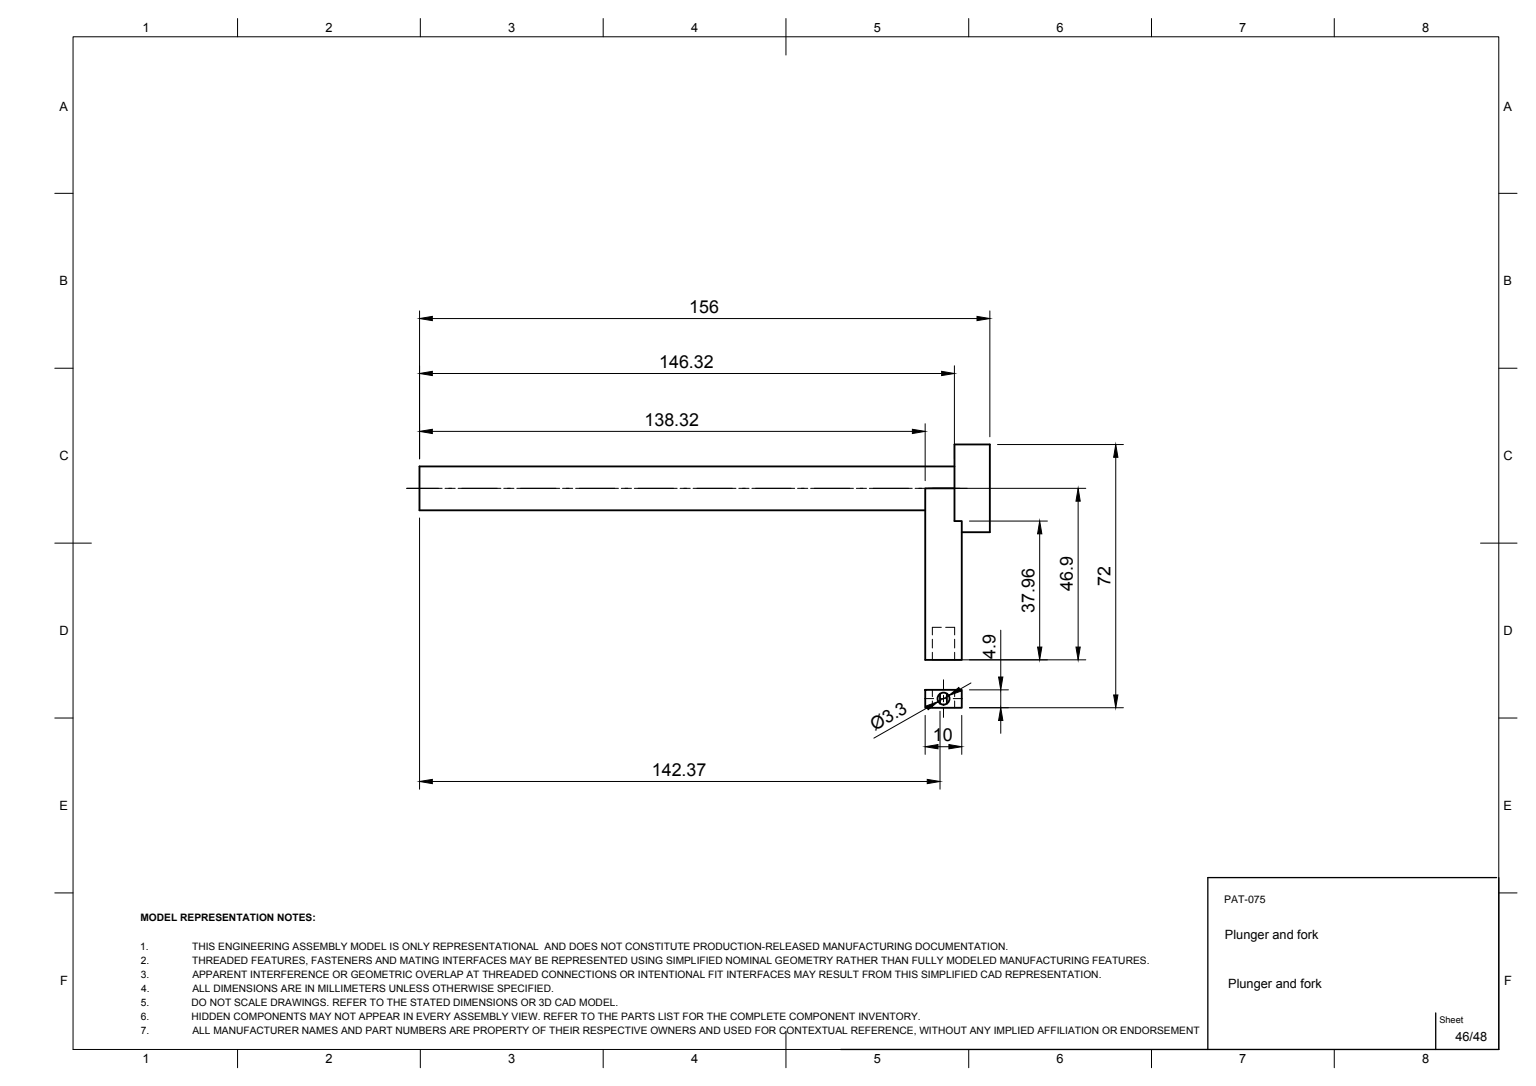
ISO-10303-21;
HEADER;
/* Generated by software containing ST-Developer
 * from STEP Tools, Inc. (www.steptools.com) 
 */

FILE_DESCRIPTION(
/* description */ ('Over-Centre Plunger Toggle Clamp on Slotted Fixture Frame'),
/* implementation_level */ '2;1');

FILE_NAME(
/* name */ 
'Plunger and fork.step',
/* time_stamp */ '2026-10-28T03:23:24-07:00',
/* author */ (''),
/* organization */ (''),
/* preprocessor_version */ 'ST-DEVELOPER v20.2',
/* originating_system */ 'Autodesk Translation Framework v15.17.0.0',
/* authorisation */ '');

FILE_SCHEMA (('AUTOMOTIVE_DESIGN { 1 0 10303 214 3 1 1 }'));
ENDSEC;

DATA;
#10=MECHANICAL_DESIGN_GEOMETRIC_PRESENTATION_REPRESENTATION('',(#559,#560),#15212);
#377=B_SPLINE_CURVE_WITH_KNOTS('',3,(#14965,#14966,#14967,#14968,#14969,
#14970,#14971,#14972,#14973,#14974),.UNSPECIFIED.,.F.,.F.,(4,2,2,2,4),(0.66642709076087,
0.700624974512804,0.764181514210609,0.827738053908413,0.861935937660348),
 .UNSPECIFIED.);
#378=B_SPLINE_CURVE_WITH_KNOTS('',3,(#14982,#14983,#14984,#14985,#14986,
#14987,#14988,#14989,#14990,#14991),.UNSPECIFIED.,.F.,.F.,(4,2,2,2,4),(0.156972747953797,
0.191170631705732,0.254727171403536,0.318283711101341,0.352481594853276),
 .UNSPECIFIED.);
#467=SHAPE_REPRESENTATION_RELATIONSHIP('SRR','None',#15446,#509);
#509=ADVANCED_BREP_SHAPE_REPRESENTATION('',(#606,#607),#15208);
#559=STYLED_ITEM('',(#15733),#606);
#560=STYLED_ITEM('',(#15733),#607);
#606=MANIFOLD_SOLID_BREP('Body1',#8295);
#607=MANIFOLD_SOLID_BREP('Body2',#8296);
#776=FACE_BOUND('',#2183,.T.);
#777=FACE_BOUND('',#2199,.T.);
#778=FACE_BOUND('',#2201,.T.);
#779=FACE_BOUND('',#2206,.T.);
#780=FACE_BOUND('',#2208,.T.);
#1054=PLANE('',#9677);
#1055=PLANE('',#9678);
#1056=PLANE('',#9679);
#1057=PLANE('',#9680);
#1058=PLANE('',#9682);
#1059=PLANE('',#9683);
#1060=PLANE('',#9684);
#1061=PLANE('',#9685);
#1062=PLANE('',#9690);
#1063=PLANE('',#9695);
#1064=PLANE('',#9696);
#1065=PLANE('',#9697);
#1066=PLANE('',#9703);
#1067=PLANE('',#9707);
#1068=PLANE('',#9708);
#1069=PLANE('',#9709);
#1070=PLANE('',#9710);
#1071=PLANE('',#9711);
#1072=PLANE('',#9712);
#1529=FACE_OUTER_BOUND('',#2180,.T.);
#1530=FACE_OUTER_BOUND('',#2181,.T.);
#1531=FACE_OUTER_BOUND('',#2182,.T.);
#1532=FACE_OUTER_BOUND('',#2184,.T.);
#1533=FACE_OUTER_BOUND('',#2185,.T.);
#1534=FACE_OUTER_BOUND('',#2186,.T.);
#1535=FACE_OUTER_BOUND('',#2187,.T.);
#1536=FACE_OUTER_BOUND('',#2188,.T.);
#1537=FACE_OUTER_BOUND('',#2189,.T.);
#1538=FACE_OUTER_BOUND('',#2190,.T.);
#1539=FACE_OUTER_BOUND('',#2191,.T.);
#1540=FACE_OUTER_BOUND('',#2192,.T.);
#1541=FACE_OUTER_BOUND('',#2193,.T.);
#1542=FACE_OUTER_BOUND('',#2194,.T.);
#1543=FACE_OUTER_BOUND('',#2195,.T.);
#1544=FACE_OUTER_BOUND('',#2196,.T.);
#1545=FACE_OUTER_BOUND('',#2197,.T.);
#1546=FACE_OUTER_BOUND('',#2198,.T.);
#1547=FACE_OUTER_BOUND('',#2200,.T.);
#1548=FACE_OUTER_BOUND('',#2202,.T.);
#1549=FACE_OUTER_BOUND('',#2203,.T.);
#1550=FACE_OUTER_BOUND('',#2204,.T.);
#1551=FACE_OUTER_BOUND('',#2205,.T.);
#1552=FACE_OUTER_BOUND('',#2207,.T.);
#2180=EDGE_LOOP('',(#7437,#7438,#7439,#7440));
#2181=EDGE_LOOP('',(#7441));
#2182=EDGE_LOOP('',(#7442,#7443,#7444,#7445));
#2183=EDGE_LOOP('',(#7446));
#2184=EDGE_LOOP('',(#7447,#7448,#7449,#7450,#7451,#7452));
#2185=EDGE_LOOP('',(#7453,#7454,#7455,#7456));
#2186=EDGE_LOOP('',(#7457,#7458,#7459,#7460,#7461,#7462));
#2187=EDGE_LOOP('',(#7463,#7464,#7465,#7466));
#2188=EDGE_LOOP('',(#7467,#7468,#7469,#7470));
#2189=EDGE_LOOP('',(#7471,#7472,#7473,#7474,#7475,#7476));
#2190=EDGE_LOOP('',(#7477,#7478,#7479,#7480,#7481,#7482,#7483));
#2191=EDGE_LOOP('',(#7484,#7485,#7486,#7487,#7488,#7489,#7490));
#2192=EDGE_LOOP('',(#7491,#7492,#7493,#7494,#7495,#7496,#7497,#7498));
#2193=EDGE_LOOP('',(#7499));
#2194=EDGE_LOOP('',(#7500));
#2195=EDGE_LOOP('',(#7501,#7502));
#2196=EDGE_LOOP('',(#7503,#7504,#7505,#7506,#7507,#7508,#7509,#7510));
#2197=EDGE_LOOP('',(#7511,#7512,#7513));
#2198=EDGE_LOOP('',(#7514,#7515,#7516,#7517));
#2199=EDGE_LOOP('',(#7518,#7519,#7520,#7521));
#2200=EDGE_LOOP('',(#7522,#7523,#7524,#7525));
#2201=EDGE_LOOP('',(#7526));
#2202=EDGE_LOOP('',(#7527,#7528,#7529,#7530));
#2203=EDGE_LOOP('',(#7531,#7532,#7533,#7534));
#2204=EDGE_LOOP('',(#7535,#7536,#7537,#7538));
#2205=EDGE_LOOP('',(#7539,#7540,#7541,#7542));
#2206=EDGE_LOOP('',(#7543));
#2207=EDGE_LOOP('',(#7544,#7545,#7546,#7547));
#2208=EDGE_LOOP('',(#7548));
#2798=LINE('',#14895,#3428);
#2799=LINE('',#14901,#3429);
#2800=LINE('',#14903,#3430);
#2801=LINE('',#14905,#3431);
#2802=LINE('',#14906,#3432);
#2803=LINE('',#14909,#3433);
#2804=LINE('',#14911,#3434);
#2805=LINE('',#14913,#3435);
#2806=LINE('',#14915,#3436);
#2807=LINE('',#14916,#3437);
#2808=LINE('',#14919,#3438);
#2809=LINE('',#14923,#3439);
#2810=LINE('',#14925,#3440);
#2811=LINE('',#14927,#3441);
#2812=LINE('',#14928,#3442);
#2813=LINE('',#14932,#3443);
#2814=LINE('',#14933,#3444);
#2815=LINE('',#14934,#3445);
#2816=LINE('',#14937,#3446);
#2817=LINE('',#14939,#3447);
#2818=LINE('',#14940,#3448);
#2819=LINE('',#14946,#3449);
#2820=LINE('',#14954,#3450);
#2821=LINE('',#14961,#3451);
#2822=LINE('',#14978,#3452);
#2823=LINE('',#14993,#3453);
#2824=LINE('',#14998,#3454);
#2825=LINE('',#15003,#3455);
#2826=LINE('',#15005,#3456);
#2827=LINE('',#15007,#3457);
#2828=LINE('',#15008,#3458);
#2829=LINE('',#15012,#3459);
#2830=LINE('',#15013,#3460);
#2831=LINE('',#15014,#3461);
#2832=LINE('',#15017,#3462);
#2833=LINE('',#15018,#3463);
#2834=LINE('',#15021,#3464);
#2835=LINE('',#15022,#3465);
#2836=LINE('',#15024,#3466);
#3428=VECTOR('',#12147,0.305);
#3429=VECTOR('',#12154,1.);
#3430=VECTOR('',#12155,1.);
#3431=VECTOR('',#12156,1.);
#3432=VECTOR('',#12157,1.);
#3433=VECTOR('',#12160,1.);
#3434=VECTOR('',#12161,1.);
#3435=VECTOR('',#12162,1.);
#3436=VECTOR('',#12163,1.);
#3437=VECTOR('',#12164,1.);
#3438=VECTOR('',#12167,1.);
#3439=VECTOR('',#12172,1.);
#3440=VECTOR('',#12173,1.);
#3441=VECTOR('',#12174,1.);
#3442=VECTOR('',#12175,1.);
#3443=VECTOR('',#12178,1.);
#3444=VECTOR('',#12179,1.);
#3445=VECTOR('',#12180,1.);
#3446=VECTOR('',#12183,1.);
#3447=VECTOR('',#12184,1.);
#3448=VECTOR('',#12185,1.);
#3449=VECTOR('',#12194,0.6);
#3450=VECTOR('',#12205,1.2);
#3451=VECTOR('',#12214,1.);
#3452=VECTOR('',#12221,0.165);
#3453=VECTOR('',#12228,1.);
#3454=VECTOR('',#12233,0.305);
#3455=VECTOR('',#12238,1.);
#3456=VECTOR('',#12239,1.);
#3457=VECTOR('',#12240,1.);
#3458=VECTOR('',#12241,1.);
#3459=VECTOR('',#12244,1.);
#3460=VECTOR('',#12245,1.);
#3461=VECTOR('',#12246,1.);
#3462=VECTOR('',#12249,1.);
#3463=VECTOR('',#12250,1.);
#3464=VECTOR('',#12253,1.);
#3465=VECTOR('',#12254,1.);
#3466=VECTOR('',#12257,1.);
#3834=CIRCLE('',#9675,0.305);
#3835=CIRCLE('',#9676,0.305);
#3836=CIRCLE('',#9681,1.2);
#3837=CIRCLE('',#9686,0.6);
#3838=CIRCLE('',#9688,0.6);
#3839=CIRCLE('',#9689,0.6);
#3840=CIRCLE('',#9691,1.2);
#3841=CIRCLE('',#9692,1.2);
#3842=CIRCLE('',#9694,1.2);
#3843=CIRCLE('',#9698,0.165);
#3844=CIRCLE('',#9700,0.165);
#3845=CIRCLE('',#9701,0.165);
#3846=CIRCLE('',#9702,0.165);
#3847=CIRCLE('',#9705,0.305);
#3848=CIRCLE('',#9706,0.305);
#4486=VERTEX_POINT('',#14892);
#4487=VERTEX_POINT('',#14894);
#4488=VERTEX_POINT('',#14899);
#4489=VERTEX_POINT('',#14900);
#4490=VERTEX_POINT('',#14902);
#4491=VERTEX_POINT('',#14904);
#4492=VERTEX_POINT('',#14908);
#4493=VERTEX_POINT('',#14910);
#4494=VERTEX_POINT('',#14912);
#4495=VERTEX_POINT('',#14914);
#4496=VERTEX_POINT('',#14918);
#4497=VERTEX_POINT('',#14922);
#4498=VERTEX_POINT('',#14924);
#4499=VERTEX_POINT('',#14926);
#4500=VERTEX_POINT('',#14930);
#4501=VERTEX_POINT('',#14931);
#4502=VERTEX_POINT('',#14936);
#4503=VERTEX_POINT('',#14938);
#4504=VERTEX_POINT('',#14944);
#4505=VERTEX_POINT('',#14949);
#4506=VERTEX_POINT('',#14953);
#4507=VERTEX_POINT('',#14959);
#4508=VERTEX_POINT('',#14960);
#4509=VERTEX_POINT('',#14964);
#4510=VERTEX_POINT('',#14975);
#4511=VERTEX_POINT('',#14977);
#4512=VERTEX_POINT('',#14980);
#4513=VERTEX_POINT('',#14995);
#4514=VERTEX_POINT('',#14997);
#4515=VERTEX_POINT('',#15001);
#4516=VERTEX_POINT('',#15002);
#4517=VERTEX_POINT('',#15004);
#4518=VERTEX_POINT('',#15006);
#4519=VERTEX_POINT('',#15010);
#4520=VERTEX_POINT('',#15011);
#4521=VERTEX_POINT('',#15016);
#4522=VERTEX_POINT('',#15020);
#5479=EDGE_CURVE('',#4486,#4486,#3834,.T.);
#5480=EDGE_CURVE('',#4486,#4487,#2798,.T.);
#5481=EDGE_CURVE('',#4487,#4487,#3835,.T.);
#5482=EDGE_CURVE('',#4488,#4489,#2799,.T.);
#5483=EDGE_CURVE('',#4490,#4488,#2800,.T.);
#5484=EDGE_CURVE('',#4491,#4490,#2801,.T.);
#5485=EDGE_CURVE('',#4489,#4491,#2802,.T.);
#5486=EDGE_CURVE('',#4490,#4492,#2803,.T.);
#5487=EDGE_CURVE('',#4493,#4492,#2804,.T.);
#5488=EDGE_CURVE('',#4494,#4493,#2805,.T.);
#5489=EDGE_CURVE('',#4494,#4495,#2806,.T.);
#5490=EDGE_CURVE('',#4491,#4495,#2807,.T.);
#5491=EDGE_CURVE('',#4496,#4488,#2808,.T.);
#5492=EDGE_CURVE('',#4492,#4496,#3836,.T.);
#5493=EDGE_CURVE('',#4497,#4489,#2809,.T.);
#5494=EDGE_CURVE('',#4498,#4497,#2810,.T.);
#5495=EDGE_CURVE('',#4499,#4498,#2811,.T.);
#5496=EDGE_CURVE('',#4496,#4499,#2812,.T.);
#5497=EDGE_CURVE('',#4500,#4501,#2813,.T.);
#5498=EDGE_CURVE('',#4495,#4500,#2814,.T.);
#5499=EDGE_CURVE('',#4501,#4494,#2815,.T.);
#5500=EDGE_CURVE('',#4498,#4502,#2816,.T.);
#5501=EDGE_CURVE('',#4503,#4497,#2817,.T.);
#5502=EDGE_CURVE('',#4502,#4503,#2818,.T.);
#5503=EDGE_CURVE('',#4503,#4500,#3837,.T.);
#5504=EDGE_CURVE('',#4504,#4504,#3838,.T.);
#5505=EDGE_CURVE('',#4504,#4503,#2819,.T.);
#5506=EDGE_CURVE('',#4501,#4502,#3839,.T.);
#5507=EDGE_CURVE('',#4493,#4505,#3840,.T.);
#5508=EDGE_CURVE('',#4505,#4499,#3841,.T.);
#5509=EDGE_CURVE('',#4505,#4506,#2820,.T.);
#5510=EDGE_CURVE('',#4506,#4506,#3842,.T.);
#5511=EDGE_CURVE('',#4507,#4508,#2821,.T.);
#5512=EDGE_CURVE('',#4507,#4508,#3843,.T.);
#5513=EDGE_CURVE('',#4509,#4507,#377,.T.);
#5514=EDGE_CURVE('',#4510,#4509,#3844,.T.);
#5515=EDGE_CURVE('',#4510,#4511,#2822,.T.);
#5516=EDGE_CURVE('',#4511,#4511,#3845,.T.);
#5517=EDGE_CURVE('',#4512,#4510,#3846,.T.);
#5518=EDGE_CURVE('',#4508,#4512,#378,.T.);
#5519=EDGE_CURVE('',#4512,#4509,#2823,.T.);
#5520=EDGE_CURVE('',#4513,#4513,#3847,.T.);
#5521=EDGE_CURVE('',#4513,#4514,#2824,.T.);
#5522=EDGE_CURVE('',#4514,#4514,#3848,.T.);
#5523=EDGE_CURVE('',#4515,#4516,#2825,.T.);
#5524=EDGE_CURVE('',#4516,#4517,#2826,.T.);
#5525=EDGE_CURVE('',#4518,#4517,#2827,.T.);
#5526=EDGE_CURVE('',#4515,#4518,#2828,.T.);
#5527=EDGE_CURVE('',#4519,#4520,#2829,.T.);
#5528=EDGE_CURVE('',#4520,#4515,#2830,.T.);
#5529=EDGE_CURVE('',#4519,#4518,#2831,.T.);
#5530=EDGE_CURVE('',#4521,#4519,#2832,.T.);
#5531=EDGE_CURVE('',#4517,#4521,#2833,.T.);
#5532=EDGE_CURVE('',#4520,#4522,#2834,.T.);
#5533=EDGE_CURVE('',#4516,#4522,#2835,.T.);
#5534=EDGE_CURVE('',#4522,#4521,#2836,.T.);
#7437=ORIENTED_EDGE('',*,*,#5479,.F.);
#7438=ORIENTED_EDGE('',*,*,#5480,.T.);
#7439=ORIENTED_EDGE('',*,*,#5481,.T.);
#7440=ORIENTED_EDGE('',*,*,#5480,.F.);
#7441=ORIENTED_EDGE('',*,*,#5481,.F.);
#7442=ORIENTED_EDGE('',*,*,#5482,.F.);
#7443=ORIENTED_EDGE('',*,*,#5483,.F.);
#7444=ORIENTED_EDGE('',*,*,#5484,.F.);
#7445=ORIENTED_EDGE('',*,*,#5485,.F.);
#7446=ORIENTED_EDGE('',*,*,#5479,.T.);
#7447=ORIENTED_EDGE('',*,*,#5484,.T.);
#7448=ORIENTED_EDGE('',*,*,#5486,.T.);
#7449=ORIENTED_EDGE('',*,*,#5487,.F.);
#7450=ORIENTED_EDGE('',*,*,#5488,.F.);
#7451=ORIENTED_EDGE('',*,*,#5489,.T.);
#7452=ORIENTED_EDGE('',*,*,#5490,.F.);
#7453=ORIENTED_EDGE('',*,*,#5483,.T.);
#7454=ORIENTED_EDGE('',*,*,#5491,.F.);
#7455=ORIENTED_EDGE('',*,*,#5492,.F.);
#7456=ORIENTED_EDGE('',*,*,#5486,.F.);
#7457=ORIENTED_EDGE('',*,*,#5482,.T.);
#7458=ORIENTED_EDGE('',*,*,#5493,.F.);
#7459=ORIENTED_EDGE('',*,*,#5494,.F.);
#7460=ORIENTED_EDGE('',*,*,#5495,.F.);
#7461=ORIENTED_EDGE('',*,*,#5496,.F.);
#7462=ORIENTED_EDGE('',*,*,#5491,.T.);
#7463=ORIENTED_EDGE('',*,*,#5497,.F.);
#7464=ORIENTED_EDGE('',*,*,#5498,.F.);
#7465=ORIENTED_EDGE('',*,*,#5489,.F.);
#7466=ORIENTED_EDGE('',*,*,#5499,.F.);
#7467=ORIENTED_EDGE('',*,*,#5500,.F.);
#7468=ORIENTED_EDGE('',*,*,#5494,.T.);
#7469=ORIENTED_EDGE('',*,*,#5501,.F.);
#7470=ORIENTED_EDGE('',*,*,#5502,.F.);
#7471=ORIENTED_EDGE('',*,*,#5485,.T.);
#7472=ORIENTED_EDGE('',*,*,#5490,.T.);
#7473=ORIENTED_EDGE('',*,*,#5498,.T.);
#7474=ORIENTED_EDGE('',*,*,#5503,.F.);
#7475=ORIENTED_EDGE('',*,*,#5501,.T.);
#7476=ORIENTED_EDGE('',*,*,#5493,.T.);
#7477=ORIENTED_EDGE('',*,*,#5504,.F.);
#7478=ORIENTED_EDGE('',*,*,#5505,.T.);
#7479=ORIENTED_EDGE('',*,*,#5503,.T.);
#7480=ORIENTED_EDGE('',*,*,#5497,.T.);
#7481=ORIENTED_EDGE('',*,*,#5506,.T.);
#7482=ORIENTED_EDGE('',*,*,#5502,.T.);
#7483=ORIENTED_EDGE('',*,*,#5505,.F.);
#7484=ORIENTED_EDGE('',*,*,#5495,.T.);
#7485=ORIENTED_EDGE('',*,*,#5500,.T.);
#7486=ORIENTED_EDGE('',*,*,#5506,.F.);
#7487=ORIENTED_EDGE('',*,*,#5499,.T.);
#7488=ORIENTED_EDGE('',*,*,#5488,.T.);
#7489=ORIENTED_EDGE('',*,*,#5507,.T.);
#7490=ORIENTED_EDGE('',*,*,#5508,.T.);
#7491=ORIENTED_EDGE('',*,*,#5496,.T.);
#7492=ORIENTED_EDGE('',*,*,#5508,.F.);
#7493=ORIENTED_EDGE('',*,*,#5509,.T.);
#7494=ORIENTED_EDGE('',*,*,#5510,.T.);
#7495=ORIENTED_EDGE('',*,*,#5509,.F.);
#7496=ORIENTED_EDGE('',*,*,#5507,.F.);
#7497=ORIENTED_EDGE('',*,*,#5487,.T.);
#7498=ORIENTED_EDGE('',*,*,#5492,.T.);
#7499=ORIENTED_EDGE('',*,*,#5510,.F.);
#7500=ORIENTED_EDGE('',*,*,#5504,.T.);
#7501=ORIENTED_EDGE('',*,*,#5511,.F.);
#7502=ORIENTED_EDGE('',*,*,#5512,.T.);
#7503=ORIENTED_EDGE('',*,*,#5513,.F.);
#7504=ORIENTED_EDGE('',*,*,#5514,.F.);
#7505=ORIENTED_EDGE('',*,*,#5515,.T.);
#7506=ORIENTED_EDGE('',*,*,#5516,.F.);
#7507=ORIENTED_EDGE('',*,*,#5515,.F.);
#7508=ORIENTED_EDGE('',*,*,#5517,.F.);
#7509=ORIENTED_EDGE('',*,*,#5518,.F.);
#7510=ORIENTED_EDGE('',*,*,#5512,.F.);
#7511=ORIENTED_EDGE('',*,*,#5519,.F.);
#7512=ORIENTED_EDGE('',*,*,#5517,.T.);
#7513=ORIENTED_EDGE('',*,*,#5514,.T.);
#7514=ORIENTED_EDGE('',*,*,#5520,.F.);
#7515=ORIENTED_EDGE('',*,*,#5521,.T.);
#7516=ORIENTED_EDGE('',*,*,#5522,.F.);
#7517=ORIENTED_EDGE('',*,*,#5521,.F.);
#7518=ORIENTED_EDGE('',*,*,#5518,.T.);
#7519=ORIENTED_EDGE('',*,*,#5519,.T.);
#7520=ORIENTED_EDGE('',*,*,#5513,.T.);
#7521=ORIENTED_EDGE('',*,*,#5511,.T.);
#7522=ORIENTED_EDGE('',*,*,#5523,.T.);
#7523=ORIENTED_EDGE('',*,*,#5524,.T.);
#7524=ORIENTED_EDGE('',*,*,#5525,.F.);
#7525=ORIENTED_EDGE('',*,*,#5526,.F.);
#7526=ORIENTED_EDGE('',*,*,#5520,.T.);
#7527=ORIENTED_EDGE('',*,*,#5527,.T.);
#7528=ORIENTED_EDGE('',*,*,#5528,.T.);
#7529=ORIENTED_EDGE('',*,*,#5526,.T.);
#7530=ORIENTED_EDGE('',*,*,#5529,.F.);
#7531=ORIENTED_EDGE('',*,*,#5530,.T.);
#7532=ORIENTED_EDGE('',*,*,#5529,.T.);
#7533=ORIENTED_EDGE('',*,*,#5525,.T.);
#7534=ORIENTED_EDGE('',*,*,#5531,.T.);
#7535=ORIENTED_EDGE('',*,*,#5532,.T.);
#7536=ORIENTED_EDGE('',*,*,#5533,.F.);
#7537=ORIENTED_EDGE('',*,*,#5523,.F.);
#7538=ORIENTED_EDGE('',*,*,#5528,.F.);
#7539=ORIENTED_EDGE('',*,*,#5534,.T.);
#7540=ORIENTED_EDGE('',*,*,#5531,.F.);
#7541=ORIENTED_EDGE('',*,*,#5524,.F.);
#7542=ORIENTED_EDGE('',*,*,#5533,.T.);
#7543=ORIENTED_EDGE('',*,*,#5516,.T.);
#7544=ORIENTED_EDGE('',*,*,#5527,.F.);
#7545=ORIENTED_EDGE('',*,*,#5530,.F.);
#7546=ORIENTED_EDGE('',*,*,#5534,.F.);
#7547=ORIENTED_EDGE('',*,*,#5532,.F.);
#7548=ORIENTED_EDGE('',*,*,#5522,.T.);
#7750=CYLINDRICAL_SURFACE('',#9674,0.305);
#7751=CYLINDRICAL_SURFACE('',#9687,0.6);
#7752=CYLINDRICAL_SURFACE('',#9693,1.2);
#7753=CYLINDRICAL_SURFACE('',#9699,0.165);
#7754=CYLINDRICAL_SURFACE('',#9704,0.305);
#8201=ADVANCED_FACE('',(#1529),#7750,.F.);
#8202=ADVANCED_FACE('',(#1530),#1054,.F.);
#8203=ADVANCED_FACE('',(#1531,#776),#1055,.F.);
#8204=ADVANCED_FACE('',(#1532),#1056,.T.);
#8205=ADVANCED_FACE('',(#1533),#1057,.F.);
#8206=ADVANCED_FACE('',(#1534),#1058,.T.);
#8207=ADVANCED_FACE('',(#1535),#1059,.T.);
#8208=ADVANCED_FACE('',(#1536),#1060,.T.);
#8209=ADVANCED_FACE('',(#1537),#1061,.T.);
#8210=ADVANCED_FACE('',(#1538),#7751,.T.);
#8211=ADVANCED_FACE('',(#1539),#1062,.T.);
#8212=ADVANCED_FACE('',(#1540),#7752,.T.);
#8213=ADVANCED_FACE('',(#1541),#1063,.F.);
#8214=ADVANCED_FACE('',(#1542),#1064,.T.);
#8215=ADVANCED_FACE('',(#1543),#1065,.T.);
#8216=ADVANCED_FACE('',(#1544),#7753,.F.);
#8217=ADVANCED_FACE('',(#1545),#1066,.T.);
#8218=ADVANCED_FACE('',(#1546,#777),#7754,.F.);
#8219=ADVANCED_FACE('',(#1547,#778),#1067,.T.);
#8220=ADVANCED_FACE('',(#1548),#1068,.T.);
#8221=ADVANCED_FACE('',(#1549),#1069,.T.);
#8222=ADVANCED_FACE('',(#1550),#1070,.F.);
#8223=ADVANCED_FACE('',(#1551,#779),#1071,.T.);
#8224=ADVANCED_FACE('',(#1552,#780),#1072,.T.);
#8295=CLOSED_SHELL('',(#8201,#8202,#8203,#8204,#8205,#8206,#8207,#8208,
#8209,#8210,#8211,#8212,#8213,#8214));
#8296=CLOSED_SHELL('',(#8215,#8216,#8217,#8218,#8219,#8220,#8221,#8222,
#8223,#8224));
#9673=AXIS2_PLACEMENT_3D('',#14890,#12141,#12142);
#9674=AXIS2_PLACEMENT_3D('',#14891,#12143,#12144);
#9675=AXIS2_PLACEMENT_3D('',#14893,#12145,#12146);
#9676=AXIS2_PLACEMENT_3D('',#14896,#12148,#12149);
#9677=AXIS2_PLACEMENT_3D('',#14897,#12150,#12151);
#9678=AXIS2_PLACEMENT_3D('',#14898,#12152,#12153);
#9679=AXIS2_PLACEMENT_3D('',#14907,#12158,#12159);
#9680=AXIS2_PLACEMENT_3D('',#14917,#12165,#12166);
#9681=AXIS2_PLACEMENT_3D('',#14920,#12168,#12169);
#9682=AXIS2_PLACEMENT_3D('',#14921,#12170,#12171);
#9683=AXIS2_PLACEMENT_3D('',#14929,#12176,#12177);
#9684=AXIS2_PLACEMENT_3D('',#14935,#12181,#12182);
#9685=AXIS2_PLACEMENT_3D('',#14941,#12186,#12187);
#9686=AXIS2_PLACEMENT_3D('',#14942,#12188,#12189);
#9687=AXIS2_PLACEMENT_3D('',#14943,#12190,#12191);
#9688=AXIS2_PLACEMENT_3D('',#14945,#12192,#12193);
#9689=AXIS2_PLACEMENT_3D('',#14947,#12195,#12196);
#9690=AXIS2_PLACEMENT_3D('',#14948,#12197,#12198);
#9691=AXIS2_PLACEMENT_3D('',#14950,#12199,#12200);
#9692=AXIS2_PLACEMENT_3D('',#14951,#12201,#12202);
#9693=AXIS2_PLACEMENT_3D('',#14952,#12203,#12204);
#9694=AXIS2_PLACEMENT_3D('',#14955,#12206,#12207);
#9695=AXIS2_PLACEMENT_3D('',#14956,#12208,#12209);
#9696=AXIS2_PLACEMENT_3D('',#14957,#12210,#12211);
#9697=AXIS2_PLACEMENT_3D('',#14958,#12212,#12213);
#9698=AXIS2_PLACEMENT_3D('',#14962,#12215,#12216);
#9699=AXIS2_PLACEMENT_3D('',#14963,#12217,#12218);
#9700=AXIS2_PLACEMENT_3D('',#14976,#12219,#12220);
#9701=AXIS2_PLACEMENT_3D('',#14979,#12222,#12223);
#9702=AXIS2_PLACEMENT_3D('',#14981,#12224,#12225);
#9703=AXIS2_PLACEMENT_3D('',#14992,#12226,#12227);
#9704=AXIS2_PLACEMENT_3D('',#14994,#12229,#12230);
#9705=AXIS2_PLACEMENT_3D('',#14996,#12231,#12232);
#9706=AXIS2_PLACEMENT_3D('',#14999,#12234,#12235);
#9707=AXIS2_PLACEMENT_3D('',#15000,#12236,#12237);
#9708=AXIS2_PLACEMENT_3D('',#15009,#12242,#12243);
#9709=AXIS2_PLACEMENT_3D('',#15015,#12247,#12248);
#9710=AXIS2_PLACEMENT_3D('',#15019,#12251,#12252);
#9711=AXIS2_PLACEMENT_3D('',#15023,#12255,#12256);
#9712=AXIS2_PLACEMENT_3D('',#15025,#12258,#12259);
#12141=DIRECTION('axis',(0.,0.,1.));
#12142=DIRECTION('refdir',(1.,0.,0.));
#12143=DIRECTION('center_axis',(0.,1.,0.));
#12144=DIRECTION('ref_axis',(1.,0.,0.));
#12145=DIRECTION('center_axis',(0.,1.,0.));
#12146=DIRECTION('ref_axis',(1.,0.,0.));
#12147=DIRECTION('',(0.,1.,0.));
#12148=DIRECTION('center_axis',(0.,1.,0.));
#12149=DIRECTION('ref_axis',(1.,0.,0.));
#12150=DIRECTION('center_axis',(0.,1.,0.));
#12151=DIRECTION('ref_axis',(1.,0.,0.));
#12152=DIRECTION('center_axis',(0.,1.,0.));
#12153=DIRECTION('ref_axis',(0.,0.,1.));
#12154=DIRECTION('',(0.,0.,1.));
#12155=DIRECTION('',(-1.,0.,0.));
#12156=DIRECTION('',(0.,0.,-1.));
#12157=DIRECTION('',(1.,0.,0.));
#12158=DIRECTION('center_axis',(1.,0.,0.));
#12159=DIRECTION('ref_axis',(0.,1.,0.));
#12160=DIRECTION('',(0.,1.,0.));
#12161=DIRECTION('',(0.,0.,-1.));
#12162=DIRECTION('',(0.,-1.,0.));
#12163=DIRECTION('',(0.,0.,1.));
#12164=DIRECTION('',(0.,1.,0.));
#12165=DIRECTION('center_axis',(0.,0.,1.));
#12166=DIRECTION('ref_axis',(1.,0.,0.));
#12167=DIRECTION('',(0.,-1.,0.));
#12168=DIRECTION('center_axis',(0.,0.,-1.));
#12169=DIRECTION('ref_axis',(1.,0.,0.));
#12170=DIRECTION('center_axis',(-1.,0.,0.));
#12171=DIRECTION('ref_axis',(0.,-1.,0.));
#12172=DIRECTION('',(0.,-1.,0.));
#12173=DIRECTION('',(0.,0.,1.));
#12174=DIRECTION('',(0.,1.,0.));
#12175=DIRECTION('',(0.,0.,1.));
#12176=DIRECTION('center_axis',(0.,1.,0.));
#12177=DIRECTION('ref_axis',(-1.,0.,0.));
#12178=DIRECTION('',(0.,0.,-1.));
#12179=DIRECTION('',(-1.,0.,0.));
#12180=DIRECTION('',(1.,0.,0.));
#12181=DIRECTION('center_axis',(0.,1.,0.));
#12182=DIRECTION('ref_axis',(-1.,0.,0.));
#12183=DIRECTION('',(1.,0.,0.));
#12184=DIRECTION('',(-1.,0.,0.));
#12185=DIRECTION('',(0.,0.,1.));
#12186=DIRECTION('center_axis',(0.,0.,1.));
#12187=DIRECTION('ref_axis',(1.,0.,0.));
#12188=DIRECTION('center_axis',(0.,0.,1.));
#12189=DIRECTION('ref_axis',(1.,0.,0.));
#12190=DIRECTION('center_axis',(0.,0.,1.));
#12191=DIRECTION('ref_axis',(1.,0.,0.));
#12192=DIRECTION('center_axis',(0.,0.,1.));
#12193=DIRECTION('ref_axis',(1.,0.,0.));
#12194=DIRECTION('',(0.,0.,-1.));
#12195=DIRECTION('center_axis',(0.,0.,1.));
#12196=DIRECTION('ref_axis',(1.,0.,0.));
#12197=DIRECTION('center_axis',(0.,0.,1.));
#12198=DIRECTION('ref_axis',(1.,0.,0.));
#12199=DIRECTION('center_axis',(0.,0.,1.));
#12200=DIRECTION('ref_axis',(1.,0.,0.));
#12201=DIRECTION('center_axis',(0.,0.,1.));
#12202=DIRECTION('ref_axis',(1.,0.,0.));
#12203=DIRECTION('center_axis',(0.,0.,1.));
#12204=DIRECTION('ref_axis',(1.,0.,0.));
#12205=DIRECTION('',(0.,0.,-1.));
#12206=DIRECTION('center_axis',(0.,0.,1.));
#12207=DIRECTION('ref_axis',(1.,0.,0.));
#12208=DIRECTION('center_axis',(0.,0.,1.));
#12209=DIRECTION('ref_axis',(1.,0.,0.));
#12210=DIRECTION('center_axis',(0.,0.,1.));
#12211=DIRECTION('ref_axis',(1.,0.,0.));
#12212=DIRECTION('center_axis',(1.,0.,0.));
#12213=DIRECTION('ref_axis',(0.,0.,-1.));
#12214=DIRECTION('',(0.,1.,0.));
#12215=DIRECTION('center_axis',(1.,0.,0.));
#12216=DIRECTION('ref_axis',(0.,0.,-1.));
#12217=DIRECTION('center_axis',(1.,0.,0.));
#12218=DIRECTION('ref_axis',(0.,0.,-1.));
#12219=DIRECTION('center_axis',(1.,0.,0.));
#12220=DIRECTION('ref_axis',(0.,0.,-1.));
#12221=DIRECTION('',(1.,0.,0.));
#12222=DIRECTION('center_axis',(-1.,0.,0.));
#12223=DIRECTION('ref_axis',(0.,0.,-1.));
#12224=DIRECTION('center_axis',(1.,0.,0.));
#12225=DIRECTION('ref_axis',(0.,0.,-1.));
#12226=DIRECTION('center_axis',(1.,0.,0.));
#12227=DIRECTION('ref_axis',(0.,0.,-1.));
#12228=DIRECTION('',(0.,-1.,0.));
#12229=DIRECTION('center_axis',(0.,1.,0.));
#12230=DIRECTION('ref_axis',(1.,0.,0.));
#12231=DIRECTION('center_axis',(0.,1.,0.));
#12232=DIRECTION('ref_axis',(1.,0.,0.));
#12233=DIRECTION('',(0.,1.,0.));
#12234=DIRECTION('center_axis',(0.,-1.,0.));
#12235=DIRECTION('ref_axis',(1.,0.,0.));
#12236=DIRECTION('center_axis',(0.,-1.,0.));
#12237=DIRECTION('ref_axis',(1.,0.,0.));
#12238=DIRECTION('',(1.,0.,0.));
#12239=DIRECTION('',(0.,0.,1.));
#12240=DIRECTION('',(1.,0.,0.));
#12241=DIRECTION('',(0.,0.,1.));
#12242=DIRECTION('center_axis',(-1.,0.,0.));
#12243=DIRECTION('ref_axis',(0.,-1.,0.));
#12244=DIRECTION('',(0.,0.,-1.));
#12245=DIRECTION('',(0.,-1.,0.));
#12246=DIRECTION('',(0.,-1.,0.));
#12247=DIRECTION('center_axis',(0.,0.,1.));
#12248=DIRECTION('ref_axis',(1.,0.,0.));
#12249=DIRECTION('',(-1.,0.,0.));
#12250=DIRECTION('',(0.,1.,0.));
#12251=DIRECTION('center_axis',(0.,0.,1.));
#12252=DIRECTION('ref_axis',(1.,0.,0.));
#12253=DIRECTION('',(1.,0.,0.));
#12254=DIRECTION('',(0.,1.,0.));
#12255=DIRECTION('center_axis',(1.,0.,0.));
#12256=DIRECTION('ref_axis',(0.,1.,0.));
#12257=DIRECTION('',(0.,0.,1.));
#12258=DIRECTION('center_axis',(0.,1.,0.));
#12259=DIRECTION('ref_axis',(1.,0.,0.));
#14890=CARTESIAN_POINT('',(0.,0.,0.));
#14891=CARTESIAN_POINT('Origin',(0.,-6.1,4.668081457105));
#14892=CARTESIAN_POINT('',(-0.305,-4.69,4.668081457105));
#14893=CARTESIAN_POINT('Origin',(0.,-4.69,4.668081457105));
#14894=CARTESIAN_POINT('',(-0.305,-3.8,4.668081457105));
#14895=CARTESIAN_POINT('',(-0.305,-6.1,4.668081457105));
#14896=CARTESIAN_POINT('Origin',(0.,-3.8,4.668081457105));
#14897=CARTESIAN_POINT('Origin',(0.,-3.8,4.668081457105));
#14898=CARTESIAN_POINT('Origin',(0.,-4.69,4.668081457105));
#14899=CARTESIAN_POINT('',(-0.8,-4.69,4.16808146));
#14900=CARTESIAN_POINT('',(-0.8,-4.69,5.16808146));
#14901=CARTESIAN_POINT('',(-0.8,-4.69,4.4180814585525));
#14902=CARTESIAN_POINT('',(0.8,-4.69,4.16808146));
#14903=CARTESIAN_POINT('',(0.,-4.69,4.16808146));
#14904=CARTESIAN_POINT('',(0.8,-4.69,5.16808146));
#14905=CARTESIAN_POINT('',(0.8,-4.69,4.4180814585525));
#14906=CARTESIAN_POINT('',(0.,-4.69,5.16808146));
#14907=CARTESIAN_POINT('Origin',(0.8,-6.,4.16808146));
#14908=CARTESIAN_POINT('',(0.8,-0.894427190999916,4.16808146));
#14909=CARTESIAN_POINT('',(0.8,-6.,4.16808146));
#14910=CARTESIAN_POINT('',(0.8,-0.894427190999916,4.36808146));
#14911=CARTESIAN_POINT('',(0.8,-0.894427190999916,3.4));
#14912=CARTESIAN_POINT('',(0.8,0.,4.36808146));
#14913=CARTESIAN_POINT('',(0.8,-3.,4.36808146));
#14914=CARTESIAN_POINT('',(0.8,0.,5.16808146));
#14915=CARTESIAN_POINT('',(0.8,0.,4.16808146));
#14916=CARTESIAN_POINT('',(0.8,-6.,5.16808146));
#14917=CARTESIAN_POINT('Origin',(0.,-3.,4.16808146));
#14918=CARTESIAN_POINT('',(-0.8,-0.894427190999916,4.16808146));
#14919=CARTESIAN_POINT('',(-0.8,0.,4.16808146));
#14920=CARTESIAN_POINT('Origin',(0.,0.,4.16808146));
#14921=CARTESIAN_POINT('Origin',(-0.8,0.,4.16808146));
#14922=CARTESIAN_POINT('',(-0.8,0.,5.16808146));
#14923=CARTESIAN_POINT('',(-0.8,0.,5.16808146));
#14924=CARTESIAN_POINT('',(-0.8,0.,4.36808146));
#14925=CARTESIAN_POINT('',(-0.8,0.,4.16808146));
#14926=CARTESIAN_POINT('',(-0.8,-0.894427190999916,4.36808146));
#14927=CARTESIAN_POINT('',(-0.8,0.,4.36808146));
#14928=CARTESIAN_POINT('',(-0.8,-0.894427190999916,3.4));
#14929=CARTESIAN_POINT('Origin',(0.8,0.,4.16808146));
#14930=CARTESIAN_POINT('',(0.6,0.,5.16808146));
#14931=CARTESIAN_POINT('',(0.6,0.,4.36808146));
#14932=CARTESIAN_POINT('',(0.6,0.,4.36808146));
#14933=CARTESIAN_POINT('',(0.8,0.,5.16808146));
#14934=CARTESIAN_POINT('',(0.4,0.,4.36808146));
#14935=CARTESIAN_POINT('Origin',(0.8,0.,4.16808146));
#14936=CARTESIAN_POINT('',(-0.6,-7.34788079488412E-17,4.36808146));
#14937=CARTESIAN_POINT('',(0.4,0.,4.36808146));
#14938=CARTESIAN_POINT('',(-0.6,0.,5.16808146));
#14939=CARTESIAN_POINT('',(0.8,0.,5.16808146));
#14940=CARTESIAN_POINT('',(-0.6,0.,4.36808146));
#14941=CARTESIAN_POINT('Origin',(0.,-3.,5.16808146));
#14942=CARTESIAN_POINT('Origin',(0.,0.,5.16808146));
#14943=CARTESIAN_POINT('Origin',(0.,0.,4.36808146));
#14944=CARTESIAN_POINT('',(-0.6,-7.34788079488412E-17,19.));
#14945=CARTESIAN_POINT('Origin',(0.,0.,19.));
#14946=CARTESIAN_POINT('',(-0.6,-7.34788079488412E-17,4.36808146));
#14947=CARTESIAN_POINT('Origin',(0.,0.,4.36808146));
#14948=CARTESIAN_POINT('Origin',(0.,0.,4.36808146));
#14949=CARTESIAN_POINT('',(-1.2,-1.46957615897682E-16,4.36808146));
#14950=CARTESIAN_POINT('Origin',(0.,0.,4.36808146));
#14951=CARTESIAN_POINT('Origin',(0.,0.,4.36808146));
#14952=CARTESIAN_POINT('Origin',(0.,0.,3.4));
#14953=CARTESIAN_POINT('',(-1.2,-1.46957615897682E-16,3.4));
#14954=CARTESIAN_POINT('',(-1.2,-1.46957615897682E-16,3.4));
#14955=CARTESIAN_POINT('Origin',(0.,0.,3.4));
#14956=CARTESIAN_POINT('Origin',(0.,0.,3.4));
#14957=CARTESIAN_POINT('Origin',(0.,0.,19.));
#14958=CARTESIAN_POINT('Origin',(0.29,-5.75,4.668081457105));
#14959=CARTESIAN_POINT('',(0.29,-5.88527749258469,4.57360923896654));
#14960=CARTESIAN_POINT('',(0.29,-5.61472250741531,4.57360923896654));
#14961=CARTESIAN_POINT('',(0.29,-6.1,4.57360923896654));
#14962=CARTESIAN_POINT('Origin',(0.29,-5.75,4.668081457105));
#14963=CARTESIAN_POINT('Origin',(0.29,-5.75,4.668081457105));
#14964=CARTESIAN_POINT('',(0.29,-5.88527749258469,4.76255367524346));
#14965=CARTESIAN_POINT('Ctrl Pts',(0.29,-5.88527749258469,4.76255367524346));
#14966=CARTESIAN_POINT('Ctrl Pts',(0.293078111442152,-5.89187616839667,
4.75310484112255));
#14967=CARTESIAN_POINT('Ctrl Pts',(0.295928845896546,-5.89761208817693,
4.7427508396533));
#14968=CARTESIAN_POINT('Ctrl Pts',(0.302593996394854,-5.91067507972101,
4.71157336496124));
#14969=CARTESIAN_POINT('Ctrl Pts',(0.305,-5.915,4.6892669703376));
#14970=CARTESIAN_POINT('Ctrl Pts',(0.305,-5.915,4.6468959438724));
#14971=CARTESIAN_POINT('Ctrl Pts',(0.302593996394854,-5.91067507972101,
4.62458954924876));
#14972=CARTESIAN_POINT('Ctrl Pts',(0.295928845896546,-5.89761208817693,
4.5934120745567));
#14973=CARTESIAN_POINT('Ctrl Pts',(0.293078111442152,-5.89187616839667,
4.58305807308745));
#14974=CARTESIAN_POINT('Ctrl Pts',(0.29,-5.88527749258469,4.57360923896654));
#14975=CARTESIAN_POINT('',(0.29,-5.75,4.833081457105));
#14976=CARTESIAN_POINT('Origin',(0.29,-5.75,4.668081457105));
#14977=CARTESIAN_POINT('',(0.8,-5.75,4.833081457105));
#14978=CARTESIAN_POINT('',(0.29,-5.75,4.833081457105));
#14979=CARTESIAN_POINT('Origin',(0.8,-5.75,4.668081457105));
#14980=CARTESIAN_POINT('',(0.29,-5.61472250741531,4.76255367524346));
#14981=CARTESIAN_POINT('Origin',(0.29,-5.75,4.668081457105));
#14982=CARTESIAN_POINT('Ctrl Pts',(0.29,-5.61472250741531,4.57360923896654));
#14983=CARTESIAN_POINT('Ctrl Pts',(0.293078111442152,-5.60812383160333,
4.58305807308745));
#14984=CARTESIAN_POINT('Ctrl Pts',(0.295928845896546,-5.60238791182307,
4.5934120745567));
#14985=CARTESIAN_POINT('Ctrl Pts',(0.302593996394854,-5.58932492027899,
4.62458954924876));
#14986=CARTESIAN_POINT('Ctrl Pts',(0.305,-5.585,4.6468959438724));
#14987=CARTESIAN_POINT('Ctrl Pts',(0.305,-5.585,4.6892669703376));
#14988=CARTESIAN_POINT('Ctrl Pts',(0.302593996394854,-5.58932492027899,
4.71157336496124));
#14989=CARTESIAN_POINT('Ctrl Pts',(0.295928845896546,-5.60238791182307,
4.7427508396533));
#14990=CARTESIAN_POINT('Ctrl Pts',(0.293078111442152,-5.60812383160333,
4.75310484112255));
#14991=CARTESIAN_POINT('Ctrl Pts',(0.29,-5.61472250741531,4.76255367524346));
#14992=CARTESIAN_POINT('Origin',(0.29,-5.75,4.668081457105));
#14993=CARTESIAN_POINT('',(0.29,-6.1,4.76255367524346));
#14994=CARTESIAN_POINT('Origin',(0.,-6.1,4.668081457105));
#14995=CARTESIAN_POINT('',(-0.305,-6.,4.668081457105));
#14996=CARTESIAN_POINT('Origin',(0.,-6.,4.668081457105));
#14997=CARTESIAN_POINT('',(-0.305,-5.51,4.668081457105));
#14998=CARTESIAN_POINT('',(-0.305,-6.1,4.668081457105));
#14999=CARTESIAN_POINT('Origin',(0.,-5.51,4.668081457105));
#15000=CARTESIAN_POINT('Origin',(-0.8,-6.,4.16808146));
#15001=CARTESIAN_POINT('',(-0.8,-6.,4.16808146));
#15002=CARTESIAN_POINT('',(0.8,-6.,4.16808146));
#15003=CARTESIAN_POINT('',(-0.8,-6.,4.16808146));
#15004=CARTESIAN_POINT('',(0.8,-6.,5.16808146));
#15005=CARTESIAN_POINT('',(0.8,-6.,4.16808146));
#15006=CARTESIAN_POINT('',(-0.8,-6.,5.16808146));
#15007=CARTESIAN_POINT('',(-0.8,-6.,5.16808146));
#15008=CARTESIAN_POINT('',(-0.8,-6.,4.16808146));
#15009=CARTESIAN_POINT('Origin',(-0.8,0.,4.16808146));
#15010=CARTESIAN_POINT('',(-0.8,-5.51,5.16808146));
#15011=CARTESIAN_POINT('',(-0.8,-5.51,4.16808146));
#15012=CARTESIAN_POINT('',(-0.8,-5.51,4.4180814585525));
#15013=CARTESIAN_POINT('',(-0.8,0.,4.16808146));
#15014=CARTESIAN_POINT('',(-0.8,0.,5.16808146));
#15015=CARTESIAN_POINT('Origin',(0.,-3.,5.16808146));
#15016=CARTESIAN_POINT('',(0.8,-5.51,5.16808146));
#15017=CARTESIAN_POINT('',(0.,-5.51,5.16808146));
#15018=CARTESIAN_POINT('',(0.8,-6.,5.16808146));
#15019=CARTESIAN_POINT('Origin',(0.,-3.,4.16808146));
#15020=CARTESIAN_POINT('',(0.8,-5.51,4.16808146));
#15021=CARTESIAN_POINT('',(0.,-5.51,4.16808146));
#15022=CARTESIAN_POINT('',(0.8,-6.,4.16808146));
#15023=CARTESIAN_POINT('Origin',(0.8,-6.,4.16808146));
#15024=CARTESIAN_POINT('',(0.8,-5.51,4.4180814585525));
#15025=CARTESIAN_POINT('Origin',(0.,-5.51,4.668081457105));
#15158=UNCERTAINTY_MEASURE_WITH_UNIT(LENGTH_MEASURE(0.001),#15213,
'DISTANCE_ACCURACY_VALUE',
'Maximum model space distance between geometric entities at asserted c
onnectivities');
#15162=UNCERTAINTY_MEASURE_WITH_UNIT(LENGTH_MEASURE(0.001),#15213,
'DISTANCE_ACCURACY_VALUE',
'Maximum model space distance between geometric entities at asserted c
onnectivities');
#15208=(
GEOMETRIC_REPRESENTATION_CONTEXT(3)
GLOBAL_UNCERTAINTY_ASSIGNED_CONTEXT((#15158))
GLOBAL_UNIT_ASSIGNED_CONTEXT((#15213,#15215,#15216))
REPRESENTATION_CONTEXT('','3D')
);
#15212=(
GEOMETRIC_REPRESENTATION_CONTEXT(3)
GLOBAL_UNCERTAINTY_ASSIGNED_CONTEXT((#15162))
GLOBAL_UNIT_ASSIGNED_CONTEXT((#15213,#15215,#15216))
REPRESENTATION_CONTEXT('','3D')
);
#15213=(
LENGTH_UNIT()
NAMED_UNIT(*)
SI_UNIT(.CENTI.,.METRE.)
);
#15215=(
NAMED_UNIT(*)
PLANE_ANGLE_UNIT()
SI_UNIT($,.RADIAN.)
);
#15216=(
NAMED_UNIT(*)
SI_UNIT($,.STERADIAN.)
SOLID_ANGLE_UNIT()
);
#15262=SHAPE_DEFINITION_REPRESENTATION(#15389,#15446);
#15389=PRODUCT_DEFINITION_SHAPE('',$,#15496);
#15446=SHAPE_REPRESENTATION('',(#9673),#15208);
#15450=PRODUCT_DEFINITION_CONTEXT('part definition',#15599,'design');
#15496=PRODUCT_DEFINITION('Plunger and fork','Plunger and fork',#15545,
#15450);
#15545=PRODUCT_DEFINITION_FORMATION('',$,#15646);
#15599=APPLICATION_CONTEXT(
'Core Data for Automotive Mechanical Design Process');
#15600=PRODUCT_CONTEXT('part definition',#15599,'mechanical');
#15646=PRODUCT('Plunger and fork','Plunger and fork','Plunger and fork',
(#15600));
#15727=COLOUR_RGB('Off White',0.89,0.88,0.83);
#15728=FILL_AREA_STYLE_COLOUR('',#15727);
#15729=FILL_AREA_STYLE('',(#15728));
#15730=SURFACE_STYLE_FILL_AREA(#15729);
#15731=SURFACE_SIDE_STYLE('',(#15730));
#15732=SURFACE_STYLE_USAGE(.BOTH.,#15731);
#15733=PRESENTATION_STYLE_ASSIGNMENT((#15732));
ENDSEC;
END-ISO-10303-21;
